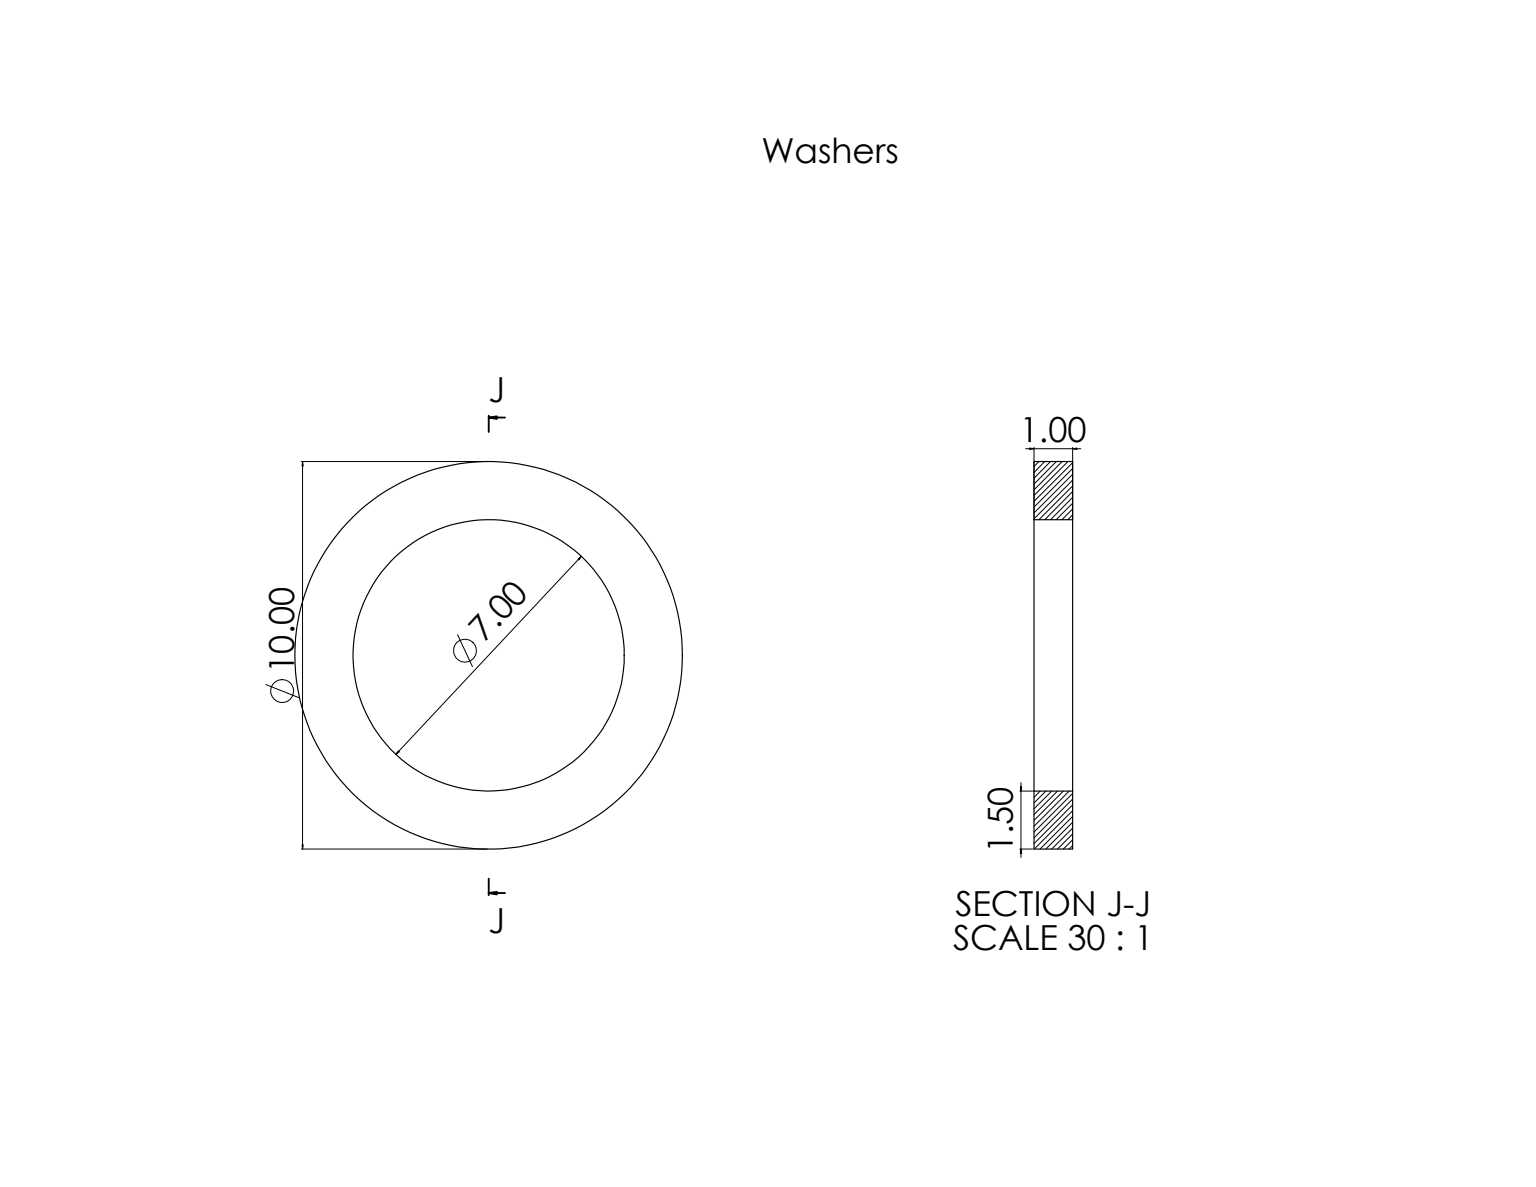
ISO-10303-21;
HEADER;
FILE_DESCRIPTION (('STEP AP214'),
    '1' );
FILE_NAME ('Washers.step',
    '2026-10-25T21:42:00',
    ( '' ),
    ( '' ),
    'SwSTEP 2.0',
    'SolidWorks 2025',
    '' );
FILE_SCHEMA (( 'AUTOMOTIVE_DESIGN' ));
ENDSEC;

DATA;
#229=ADVANCED_FACE ( 'NONE', ( #9847, #38761 ), #26005, .T. ) ;
#757=VECTOR ( 'NONE', #17426, 1000.000000000000000 ) ;
#767=AXIS2_PLACEMENT_3D ( 'NONE', #9830, #26400, #25572 ) ;
#1176=EDGE_CURVE ( 'NONE', #4829, #36324, #22704, .T. ) ;
#1274=DIRECTION ( 'NONE',  ( -1.000000000000000000, 0.000000000000000000, 0.000000000000000000 ) ) ;
#2043=VERTEX_POINT ( 'NONE', #7439 ) ;
#2102=ADVANCED_FACE ( 'NONE', ( #26803 ), #36791, .T. ) ;
#2221=EDGE_CURVE ( 'NONE', #36324, #28318, #25883, .T. ) ;
#2609=DIRECTION ( 'NONE',  ( 1.000000000000000000, 0.000000000000000000, -0.000000000000000000 ) ) ;
#3093=CYLINDRICAL_SURFACE ( 'NONE', #20648, 3.500000000000005329 ) ;
#3243=CARTESIAN_POINT ( 'NONE',  ( 3.500000000000005329, 17.49999999999998934, -76.99999999999998579 ) ) ;
#4148=( NAMED_UNIT ( * ) SI_UNIT ( $, .STERADIAN. ) SOLID_ANGLE_UNIT ( ) );
#4192=CARTESIAN_POINT ( 'NONE',  ( 3.500000000000005329, 17.49999999999998934, -76.99999999999998579 ) ) ;
#4365=SHAPE_REPRESENTATION_RELATIONSHIP ( 'NONE' , 'NONE' ,  #7898, #35064 ) ;
#4437=AXIS2_PLACEMENT_3D ( 'NONE', #24954, #31321, #17935 ) ;
#4829=VERTEX_POINT ( 'NONE', #15622 ) ;
#4847=ADVANCED_FACE ( 'NONE', ( #19430, #38574 ), #16051, .F. ) ;
#5908=EDGE_CURVE ( 'NONE', #26418, #11214, #23273, .T. ) ;
#6845=EDGE_CURVE ( 'NONE', #22985, #9428, #32462, .T. ) ;
#6924=AXIS2_PLACEMENT_3D ( 'NONE', #26514, #30326, #23323 ) ;
#7151=DIRECTION ( 'NONE',  ( -0.000000000000000000, -0.000000000000000000, -1.000000000000000000 ) ) ;
#7439=CARTESIAN_POINT ( 'NONE',  ( 5.000000000000005329, 17.49999999999998934, -77.99999999999998579 ) ) ;
#7670=ORIENTED_EDGE ( 'NONE', *, *, #2221, .T. ) ;
#7898=SHAPE_REPRESENTATION ( 'Washers', ( #40442 ), #8523 ) ;
#8013=LINE ( 'NONE', #4192, #18581 ) ;
#8180=ORIENTED_EDGE ( 'NONE', *, *, #1176, .T. ) ;
#8468=AXIS2_PLACEMENT_3D ( 'NONE', #31558, #18176, #24565 ) ;
#8507=EDGE_CURVE ( 'NONE', #26418, #9428, #8013, .T. ) ;
#8523=( GEOMETRIC_REPRESENTATION_CONTEXT ( 3 ) GLOBAL_UNCERTAINTY_ASSIGNED_CONTEXT ( ( #9296 ) ) GLOBAL_UNIT_ASSIGNED_CONTEXT ( ( #22157, #9179, #4148 ) ) REPRESENTATION_CONTEXT ( 'NONE', 'WORKASPACE' ) );
#8634=ORIENTED_EDGE ( 'NONE', *, *, #33974, .T. ) ;
#8872=PRODUCT ( 'Washers', 'Washers', '', ( #26496 ) ) ;
#9067=CLOSED_SHELL ( 'NONE', ( #39320, #2102, #229, #4847, #18748, #40205 ) ) ;
#9094=( NAMED_UNIT ( * ) SI_UNIT ( $, .STERADIAN. ) SOLID_ANGLE_UNIT ( ) );
#9099=AXIS2_PLACEMENT_3D ( 'NONE', #19927, #32479, #29072 ) ;
#9179=( NAMED_UNIT ( * ) PLANE_ANGLE_UNIT ( ) SI_UNIT ( $, .RADIAN. ) );
#9296=UNCERTAINTY_MEASURE_WITH_UNIT (LENGTH_MEASURE( 1.000000000000000082E-05 ), #22157, 'distance_accuracy_value', 'NONE');
#9428=VERTEX_POINT ( 'NONE', #13558 ) ;
#9504=DIRECTION ( 'NONE',  ( -0.000000000000000000, -0.000000000000000000, -1.000000000000000000 ) ) ;
#9520=( NAMED_UNIT ( * ) PLANE_ANGLE_UNIT ( ) SI_UNIT ( $, .RADIAN. ) );
#9632=DIRECTION ( 'NONE',  ( 0.000000000000000000, 0.000000000000000000, 1.000000000000000000 ) ) ;
#9830=CARTESIAN_POINT ( 'NONE',  ( 0.000000000000000000, 17.49999999999998934, -76.99999999999998579 ) ) ;
#9847=FACE_OUTER_BOUND ( 'NONE', #35699, .T. ) ;
#9904=CARTESIAN_POINT ( 'NONE',  ( 0.000000000000000000, 17.49999999999998934, -76.99999999999998579 ) ) ;
#10179=MECHANICAL_DESIGN_GEOMETRIC_PRESENTATION_REPRESENTATION('',(#18314),#40056);
#10326=SHAPE_DEFINITION_REPRESENTATION ( #16985, #7898 ) ;
#10827=ORIENTED_EDGE ( 'NONE', *, *, #6845, .F. ) ;
#11131=CARTESIAN_POINT ( 'NONE',  ( 0.000000000000000000, 0.000000000000000000, 0.000000000000000000 ) ) ;
#11172=AXIS2_PLACEMENT_3D ( 'NONE', #33163, #29764, #1274 ) ;
#11214=VERTEX_POINT ( 'NONE', #36601 ) ;
#11628=CIRCLE ( 'NONE', #767, 3.500000000000005329 ) ;
#11661=ORIENTED_EDGE ( 'NONE', *, *, #19221, .T. ) ;
#11745=DIRECTION ( 'NONE',  ( 1.000000000000000000, 0.000000000000000000, 0.000000000000000000 ) ) ;
#12421=DIRECTION ( 'NONE',  ( 0.000000000000000000, 0.000000000000000000, 1.000000000000000000 ) ) ;
#12467=EDGE_LOOP ( 'NONE', ( #38050, #18635, #8634, #37415 ) ) ;
#12474=CARTESIAN_POINT ( 'NONE',  ( -5.000000000000005329, 17.49999999999998934, -76.99999999999998579 ) ) ;
#12622=ORIENTED_EDGE ( 'NONE', *, *, #8507, .T. ) ;
#12741=EDGE_LOOP ( 'NONE', ( #39724, #12622, #10827, #28040 ) ) ;
#13558=CARTESIAN_POINT ( 'NONE',  ( 3.500000000000005329, 17.49999999999998934, -77.99999999999998579 ) ) ;
#13924=ORIENTED_EDGE ( 'NONE', *, *, #6845, .T. ) ;
#14348=AXIS2_PLACEMENT_3D ( 'NONE', #32611, #32205, #29004 ) ;
#15504=ORIENTED_EDGE ( 'NONE', *, *, #20726, .T. ) ;
#15622=CARTESIAN_POINT ( 'NONE',  ( 5.000000000000005329, 17.49999999999998934, -76.99999999999998579 ) ) ;
#16051=PLANE ( 'NONE',  #22569 ) ;
#16086=DIRECTION ( 'NONE',  ( -0.000000000000000000, -0.000000000000000000, -1.000000000000000000 ) ) ;
#16137=CARTESIAN_POINT ( 'NONE',  ( -5.000000000000005329, 17.49999999999998934, -77.99999999999998579 ) ) ;
#16899=DIRECTION ( 'NONE',  ( -1.000000000000000000, 0.000000000000000000, 0.000000000000000000 ) ) ;
#16985=PRODUCT_DEFINITION_SHAPE ( 'NONE', 'NONE',  #22621 ) ;
#17345=CIRCLE ( 'NONE', #4437, 5.000000000000005329 ) ;
#17426=DIRECTION ( 'NONE',  ( -0.000000000000000000, -0.000000000000000000, -1.000000000000000000 ) ) ;
#17556=CARTESIAN_POINT ( 'NONE',  ( 5.000000000000005329, 17.49999999999998934, -76.99999999999998579 ) ) ;
#17747=CIRCLE ( 'NONE', #14348, 5.000000000000005329 ) ;
#17935=DIRECTION ( 'NONE',  ( 1.000000000000000000, 0.000000000000000000, 0.000000000000000000 ) ) ;
#18140=CARTESIAN_POINT ( 'NONE',  ( 0.000000000000000000, 17.49999999999998934, -76.99999999999998579 ) ) ;
#18176=DIRECTION ( 'NONE',  ( -0.000000000000000000, -0.000000000000000000, -1.000000000000000000 ) ) ;
#18314=STYLED_ITEM('',(#42159),#23783);
#18581=VECTOR ( 'NONE', #20789, 1000.000000000000000 ) ;
#18599=CARTESIAN_POINT ( 'NONE',  ( -3.500000000000005329, 17.49999999999998934, -77.99999999999998579 ) ) ;
#18635=ORIENTED_EDGE ( 'NONE', *, *, #22824, .T. ) ;
#18701=PRODUCT_DEFINITION_FORMATION_WITH_SPECIFIED_SOURCE ( 'ANY', '', #8872, .NOT_KNOWN. ) ;
#18748=ADVANCED_FACE ( 'NONE', ( #35661 ), #36278, .T. ) ;
#18979=ORIENTED_EDGE ( 'NONE', *, *, #19221, .F. ) ;
#19221=EDGE_CURVE ( 'NONE', #36324, #4829, #17747, .T. ) ;
#19430=FACE_OUTER_BOUND ( 'NONE', #35216, .T. ) ;
#19583=EDGE_CURVE ( 'NONE', #11214, #26418, #11628, .T. ) ;
#19927=CARTESIAN_POINT ( 'NONE',  ( 0.000000000000000000, 17.49999999999998934, -76.99999999999998579 ) ) ;
#20121=DIRECTION ( 'NONE',  ( -1.000000000000000000, 0.000000000000000000, 0.000000000000000000 ) ) ;
#20648=AXIS2_PLACEMENT_3D ( 'NONE', #9904, #16086, #16899 ) ;
#20726=EDGE_CURVE ( 'NONE', #9428, #22985, #27964, .T. ) ;
#20789=DIRECTION ( 'NONE',  ( -0.000000000000000000, -0.000000000000000000, -1.000000000000000000 ) ) ;
#20814=DIRECTION ( 'NONE',  ( 0.000000000000000000, 0.000000000000000000, 1.000000000000000000 ) ) ;
#21030=VECTOR ( 'NONE', #30521, 1000.000000000000000 ) ;
#21153=FACE_OUTER_BOUND ( 'NONE', #21858, .T. ) ;
#21858=EDGE_LOOP ( 'NONE', ( #35741, #23601, #37665, #23518 ) ) ;
#22157=( LENGTH_UNIT ( ) NAMED_UNIT ( * ) SI_UNIT ( .MILLI., .METRE. ) );
#22569=AXIS2_PLACEMENT_3D ( 'NONE', #22620, #12421, #28581 ) ;
#22620=CARTESIAN_POINT ( 'NONE',  ( 0.000000000000000000, 17.49999999999998934, -77.99999999999998579 ) ) ;
#22621=PRODUCT_DEFINITION ( 'UNKNOWN', '', #18701, #26720 ) ;
#22704=CIRCLE ( 'NONE', #9099, 5.000000000000005329 ) ;
#22727=VECTOR ( 'NONE', #9504, 1000.000000000000000 ) ;
#22824=EDGE_CURVE ( 'NONE', #4829, #2043, #33506, .T. ) ;
#22985=VERTEX_POINT ( 'NONE', #18599 ) ;
#23273=CIRCLE ( 'NONE', #28008, 3.500000000000005329 ) ;
#23323=DIRECTION ( 'NONE',  ( 1.000000000000000000, 0.000000000000000000, 0.000000000000000000 ) ) ;
#23518=ORIENTED_EDGE ( 'NONE', *, *, #20726, .F. ) ;
#23576=ORIENTED_EDGE ( 'NONE', *, *, #22824, .F. ) ;
#23601=ORIENTED_EDGE ( 'NONE', *, *, #5908, .T. ) ;
#23643=AXIS2_PLACEMENT_3D ( 'NONE', #34512, #30915, #34097 ) ;
#23783=MANIFOLD_SOLID_BREP ( 'Boss-Extrude15', #9067 ) ;
#24112=DIRECTION ( 'NONE',  ( 0.000000000000000000, 0.000000000000000000, 1.000000000000000000 ) ) ;
#24565=DIRECTION ( 'NONE',  ( -1.000000000000000000, 0.000000000000000000, 0.000000000000000000 ) ) ;
#24954=CARTESIAN_POINT ( 'NONE',  ( 0.000000000000000000, 17.49999999999998934, -77.99999999999998579 ) ) ;
#25060=( LENGTH_UNIT ( ) NAMED_UNIT ( * ) SI_UNIT ( .MILLI., .METRE. ) );
#25219=AXIS2_PLACEMENT_3D ( 'NONE', #36065, #7151, #20121 ) ;
#25572=DIRECTION ( 'NONE',  ( 1.000000000000000000, 0.000000000000000000, 0.000000000000000000 ) ) ;
#25756=CIRCLE ( 'NONE', #34580, 5.000000000000005329 ) ;
#25883=LINE ( 'NONE', #36064, #22727 ) ;
#26005=PLANE ( 'NONE',  #41014 ) ;
#26400=DIRECTION ( 'NONE',  ( 0.000000000000000000, 0.000000000000000000, 1.000000000000000000 ) ) ;
#26418=VERTEX_POINT ( 'NONE', #3243 ) ;
#26496=PRODUCT_CONTEXT ( 'NONE', #26917, 'mechanical' ) ;
#26514=CARTESIAN_POINT ( 'NONE',  ( 0.000000000000000000, 17.49999999999998934, -77.99999999999998579 ) ) ;
#26720=PRODUCT_DEFINITION_CONTEXT ( 'detailed design', #27712, 'design' ) ;
#26803=FACE_OUTER_BOUND ( 'NONE', #12467, .T. ) ;
#26917=APPLICATION_CONTEXT ( 'automotive_design' ) ;
#27712=APPLICATION_CONTEXT ( 'automotive_design' ) ;
#27839=ORIENTED_EDGE ( 'NONE', *, *, #19583, .F. ) ;
#27964=CIRCLE ( 'NONE', #6924, 3.500000000000005329 ) ;
#28008=AXIS2_PLACEMENT_3D ( 'NONE', #18140, #31110, #11745 ) ;
#28040=ORIENTED_EDGE ( 'NONE', *, *, #29297, .F. ) ;
#28318=VERTEX_POINT ( 'NONE', #16137 ) ;
#28581=DIRECTION ( 'NONE',  ( 1.000000000000000000, 0.000000000000000000, -0.000000000000000000 ) ) ;
#28624=EDGE_LOOP ( 'NONE', ( #13924, #15504 ) ) ;
#28727=ORIENTED_EDGE ( 'NONE', *, *, #33974, .F. ) ;
#29004=DIRECTION ( 'NONE',  ( 1.000000000000000000, 0.000000000000000000, 0.000000000000000000 ) ) ;
#29072=DIRECTION ( 'NONE',  ( 1.000000000000000000, 0.000000000000000000, 0.000000000000000000 ) ) ;
#29297=EDGE_CURVE ( 'NONE', #11214, #22985, #36769, .T. ) ;
#29573=ORIENTED_EDGE ( 'NONE', *, *, #32699, .F. ) ;
#29764=DIRECTION ( 'NONE',  ( -0.000000000000000000, -0.000000000000000000, -1.000000000000000000 ) ) ;
#30326=DIRECTION ( 'NONE',  ( 0.000000000000000000, 0.000000000000000000, 1.000000000000000000 ) ) ;
#30521=DIRECTION ( 'NONE',  ( -0.000000000000000000, -0.000000000000000000, -1.000000000000000000 ) ) ;
#30594=CARTESIAN_POINT ( 'NONE',  ( -3.500000000000005329, 17.49999999999998934, -76.99999999999998579 ) ) ;
#30915=DIRECTION ( 'NONE',  ( 0.000000000000000000, 0.000000000000000000, 1.000000000000000000 ) ) ;
#31110=DIRECTION ( 'NONE',  ( 0.000000000000000000, 0.000000000000000000, 1.000000000000000000 ) ) ;
#31321=DIRECTION ( 'NONE',  ( 0.000000000000000000, 0.000000000000000000, 1.000000000000000000 ) ) ;
#31558=CARTESIAN_POINT ( 'NONE',  ( 0.000000000000000000, 17.49999999999998934, -76.99999999999998579 ) ) ;
#31827=UNCERTAINTY_MEASURE_WITH_UNIT (LENGTH_MEASURE( 1.000000000000000082E-05 ), #25060, 'distance_accuracy_value', 'NONE');
#32205=DIRECTION ( 'NONE',  ( 0.000000000000000000, 0.000000000000000000, 1.000000000000000000 ) ) ;
#32462=CIRCLE ( 'NONE', #23643, 3.500000000000005329 ) ;
#32479=DIRECTION ( 'NONE',  ( 0.000000000000000000, 0.000000000000000000, 1.000000000000000000 ) ) ;
#32611=CARTESIAN_POINT ( 'NONE',  ( 0.000000000000000000, 17.49999999999998934, -76.99999999999998579 ) ) ;
#32699=EDGE_CURVE ( 'NONE', #28318, #2043, #25756, .T. ) ;
#33005=ORIENTED_EDGE ( 'NONE', *, *, #5908, .F. ) ;
#33163=CARTESIAN_POINT ( 'NONE',  ( 0.000000000000000000, 17.49999999999998934, -76.99999999999998579 ) ) ;
#33506=LINE ( 'NONE', #17556, #21030 ) ;
#33787=DIRECTION ( 'NONE',  ( 1.000000000000000000, 0.000000000000000000, 0.000000000000000000 ) ) ;
#33974=EDGE_CURVE ( 'NONE', #2043, #28318, #17345, .T. ) ;
#34097=DIRECTION ( 'NONE',  ( 1.000000000000000000, 0.000000000000000000, 0.000000000000000000 ) ) ;
#34381=EDGE_LOOP ( 'NONE', ( #27839, #33005 ) ) ;
#34512=CARTESIAN_POINT ( 'NONE',  ( 0.000000000000000000, 17.49999999999998934, -77.99999999999998579 ) ) ;
#34580=AXIS2_PLACEMENT_3D ( 'NONE', #37186, #20814, #33787 ) ;
#35064=ADVANCED_BREP_SHAPE_REPRESENTATION ( '', ( #23783, #40442 ), #8523 ) ;
#35209=EDGE_LOOP ( 'NONE', ( #23576, #18979, #7670, #40874 ) ) ;
#35216=EDGE_LOOP ( 'NONE', ( #29573, #28727 ) ) ;
#35570=CARTESIAN_POINT ( 'NONE',  ( 0.000000000000000000, 17.49999999999998934, -76.99999999999998579 ) ) ;
#35661=FACE_OUTER_BOUND ( 'NONE', #35209, .T. ) ;
#35699=EDGE_LOOP ( 'NONE', ( #11661, #8180 ) ) ;
#35741=ORIENTED_EDGE ( 'NONE', *, *, #8507, .F. ) ;
#36064=CARTESIAN_POINT ( 'NONE',  ( -5.000000000000005329, 17.49999999999998934, -76.99999999999998579 ) ) ;
#36065=CARTESIAN_POINT ( 'NONE',  ( 0.000000000000000000, 17.49999999999998934, -76.99999999999998579 ) ) ;
#36278=CYLINDRICAL_SURFACE ( 'NONE', #25219, 5.000000000000005329 ) ;
#36324=VERTEX_POINT ( 'NONE', #12474 ) ;
#36601=CARTESIAN_POINT ( 'NONE',  ( -3.500000000000005329, 17.49999999999998934, -76.99999999999998579 ) ) ;
#36650=DIRECTION ( 'NONE',  ( 1.000000000000000000, 0.000000000000000000, 0.000000000000000000 ) ) ;
#36769=LINE ( 'NONE', #30594, #757 ) ;
#36791=CYLINDRICAL_SURFACE ( 'NONE', #11172, 5.000000000000005329 ) ;
#37186=CARTESIAN_POINT ( 'NONE',  ( 0.000000000000000000, 17.49999999999998934, -77.99999999999998579 ) ) ;
#37415=ORIENTED_EDGE ( 'NONE', *, *, #2221, .F. ) ;
#37527=CYLINDRICAL_SURFACE ( 'NONE', #8468, 3.500000000000005329 ) ;
#37665=ORIENTED_EDGE ( 'NONE', *, *, #29297, .T. ) ;
#38050=ORIENTED_EDGE ( 'NONE', *, *, #1176, .F. ) ;
#38574=FACE_BOUND ( 'NONE', #28624, .T. ) ;
#38761=FACE_BOUND ( 'NONE', #34381, .T. ) ;
#39019=FACE_OUTER_BOUND ( 'NONE', #12741, .T. ) ;
#39320=ADVANCED_FACE ( 'NONE', ( #39019 ), #3093, .F. ) ;
#39724=ORIENTED_EDGE ( 'NONE', *, *, #19583, .T. ) ;
#40056=( GEOMETRIC_REPRESENTATION_CONTEXT ( 3 ) GLOBAL_UNCERTAINTY_ASSIGNED_CONTEXT ( ( #31827 ) ) GLOBAL_UNIT_ASSIGNED_CONTEXT ( ( #25060, #9520, #9094 ) ) REPRESENTATION_CONTEXT ( 'NONE', 'WORKASPACE' ) );
#40205=ADVANCED_FACE ( 'NONE', ( #21153 ), #37527, .F. ) ;
#40442=AXIS2_PLACEMENT_3D ( 'NONE', #11131, #24112, #36650 ) ;
#40874=ORIENTED_EDGE ( 'NONE', *, *, #32699, .T. ) ;
#41014=AXIS2_PLACEMENT_3D ( 'NONE', #35570, #9632, #2609 ) ;
#42153=COLOUR_RGB('Black',0.12,0.14,0.17);
#42154=FILL_AREA_STYLE_COLOUR('',#42153);
#42155=FILL_AREA_STYLE('',(#42154));
#42156=SURFACE_STYLE_FILL_AREA(#42155);
#42157=SURFACE_SIDE_STYLE('',(#42156));
#42158=SURFACE_STYLE_USAGE(.BOTH.,#42157);
#42159=PRESENTATION_STYLE_ASSIGNMENT((#42158));
ENDSEC;
END-ISO-10303-21;
